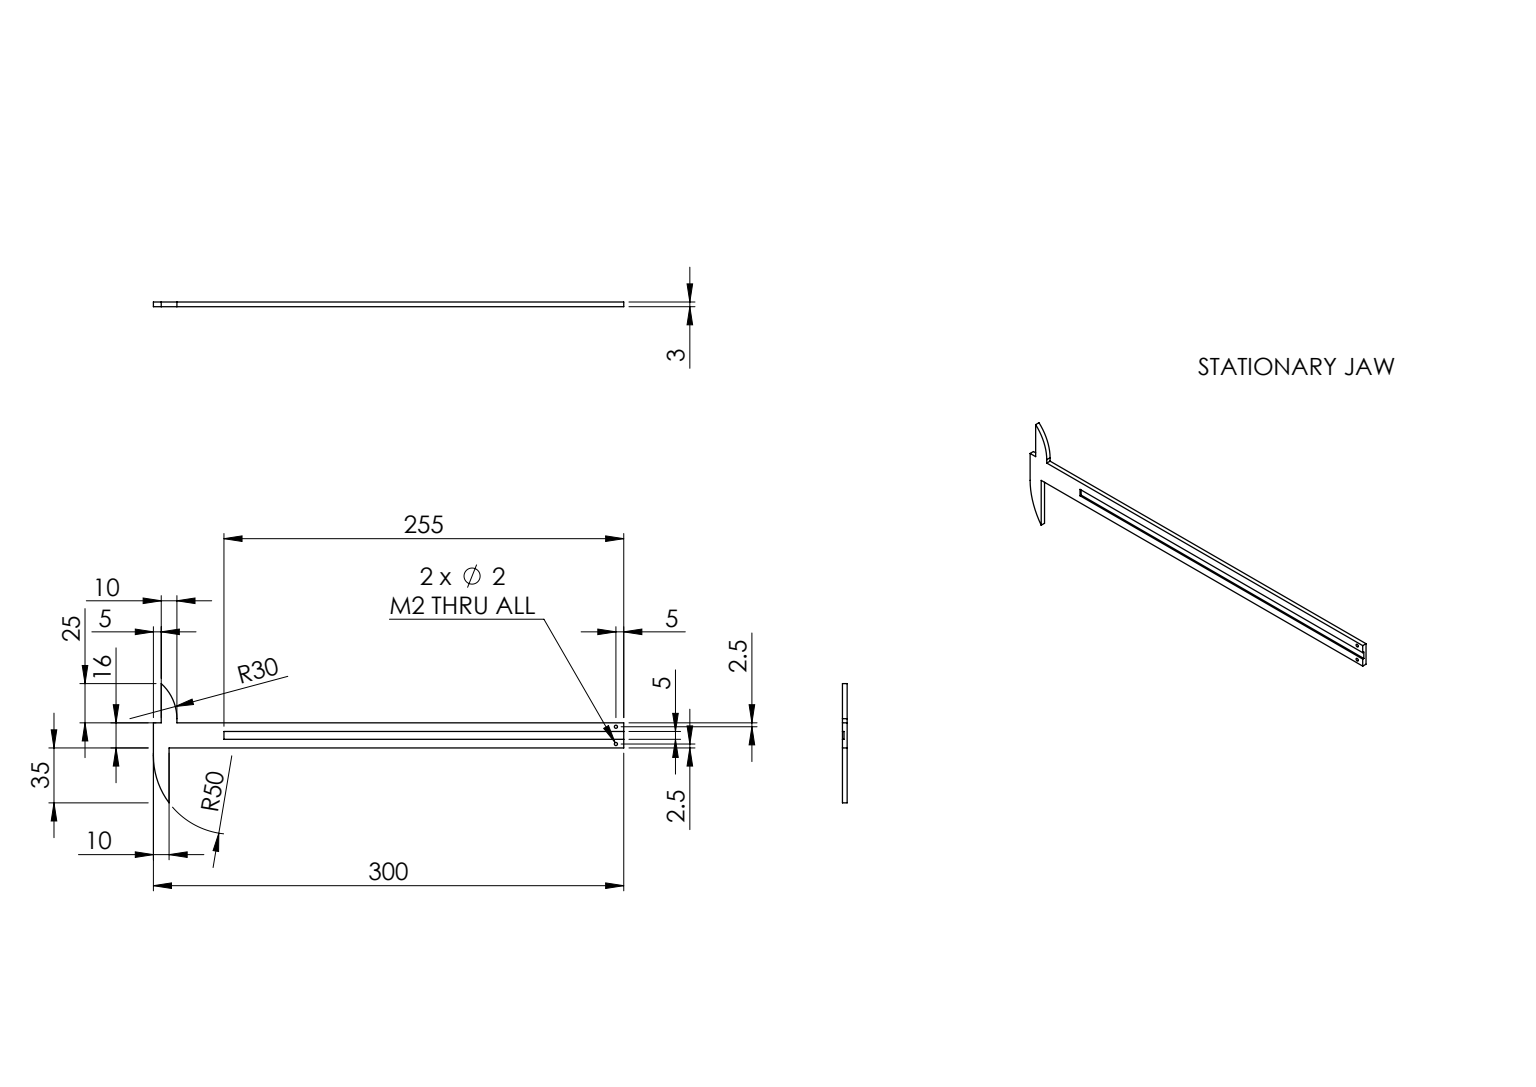
ISO-10303-21;
HEADER;
FILE_DESCRIPTION (('STEP AP214'),
    '1' );
FILE_NAME ('stationary jaw.step',
    '2026-10-27T04:40:18',
    ( '' ),
    ( '' ),
    'SwSTEP 2.0',
    'SolidWorks 2026',
    '' );
FILE_SCHEMA (( 'AUTOMOTIVE_DESIGN' ));
ENDSEC;

DATA;
#11=FACE_OUTER_BOUND ( 'NONE', #2535, .T. ) ;
#34=CARTESIAN_POINT ( 'NONE',  ( -149.9999999999999716, 8.000000000000000000, 0.000000000000000000 ) ) ;
#53=CARTESIAN_POINT ( 'NONE',  ( 144.0000000000000284, -5.500000000000000000, 3.000000000000000000 ) ) ;
#117=DIRECTION ( 'NONE',  ( 0.000000000000000000, 0.000000000000000000, 1.000000000000000000 ) ) ;
#146=EDGE_CURVE ( 'NONE', #6970, #9736, #4895, .T. ) ;
#150=VECTOR ( 'NONE', #8789, 1000.000000000000000 ) ;
#162=AXIS2_PLACEMENT_3D ( 'NONE', #9186, #3975, #9242 ) ;
#173=DIRECTION ( 'NONE',  ( -0.000000000000000000, -0.000000000000000000, 1.000000000000000000 ) ) ;
#192=VERTEX_POINT ( 'NONE', #7412 ) ;
#204=( NAMED_UNIT ( * ) PLANE_ANGLE_UNIT ( ) SI_UNIT ( $, .RADIAN. ) );
#247=ADVANCED_FACE ( 'NONE', ( #10016 ), #2398, .F. ) ;
#272=DIRECTION ( 'NONE',  ( 0.000000000000000000, 0.000000000000000000, -1.000000000000000000 ) ) ;
#276=DIRECTION ( 'NONE',  ( 1.000000000000000000, 0.000000000000000000, 0.000000000000000000 ) ) ;
#313=CARTESIAN_POINT ( 'NONE',  ( -105.0000000000000000, -2.500000000000000000, 4.000000000000000000 ) ) ;
#328=CIRCLE ( 'NONE', #5652, 1.000000000000000888 ) ;
#334=DIRECTION ( 'NONE',  ( 1.000000000000000000, 0.000000000000000000, 0.000000000000000000 ) ) ;
#362=EDGE_CURVE ( 'NONE', #4689, #5869, #2786, .T. ) ;
#386=VERTEX_POINT ( 'NONE', #1056 ) ;
#391=ORIENTED_EDGE ( 'NONE', *, *, #9319, .T. ) ;
#404=DIRECTION ( 'NONE',  ( 0.000000000000000000, 0.000000000000000000, 1.000000000000000000 ) ) ;
#406=DIRECTION ( 'NONE',  ( 1.734723475976807094E-15, -1.000000000000000000, 0.000000000000000000 ) ) ;
#407=UNCERTAINTY_MEASURE_WITH_UNIT (LENGTH_MEASURE( 1.000000000000000082E-05 ), #5246, 'distance_accuracy_value', 'NONE');
#409=EDGE_LOOP ( 'NONE', ( #9606, #6475, #9228, #1255, #10309, #5081, #6466, #4394, #2415, #6355, #391, #7202, #777, #5042 ) ) ;
#427=VERTEX_POINT ( 'NONE', #7181 ) ;
#477=CARTESIAN_POINT ( 'NONE',  ( 0.000000000000000000, -2.500000000000000000, 3.000000000000000000 ) ) ;
#478=ORIENTED_EDGE ( 'NONE', *, *, #3539, .T. ) ;
#503=ADVANCED_FACE ( 'NONE', ( #6406 ), #2069, .T. ) ;
#510=LINE ( 'NONE', #9841, #4674 ) ;
#547=AXIS2_PLACEMENT_3D ( 'NONE', #10152, #5041, #1715 ) ;
#567=CARTESIAN_POINT ( 'NONE',  ( -149.9999999999999716, 8.000000000000000000, 3.000000000000000000 ) ) ;
#573=DIRECTION ( 'NONE',  ( -0.000000000000000000, -0.000000000000000000, 1.000000000000000000 ) ) ;
#592=AXIS2_PLACEMENT_3D ( 'NONE', #10434, #7171, #272 ) ;
#599=AXIS2_PLACEMENT_3D ( 'NONE', #4517, #5230, #6973 ) ;
#604=CIRCLE ( 'NONE', #9648, 1.000000000000000888 ) ;
#667=LINE ( 'NONE', #7455, #4965 ) ;
#670=LINE ( 'NONE', #9229, #10699 ) ;
#678=AXIS2_PLACEMENT_3D ( 'NONE', #10292, #1697, #1916 ) ;
#680=DIRECTION ( 'NONE',  ( -0.000000000000000000, 1.000000000000000000, -0.000000000000000000 ) ) ;
#683=AXIS2_PLACEMENT_3D ( 'NONE', #6099, #5365, #6331 ) ;
#686=FACE_BOUND ( 'NONE', #7136, .T. ) ;
#687=CARTESIAN_POINT ( 'NONE',  ( 150.0000000000000284, -8.000000000000000000, 3.000000000000000000 ) ) ;
#725=DIRECTION ( 'NONE',  ( -1.734723475976807094E-15, 1.000000000000000000, 0.000000000000000000 ) ) ;
#727=DIRECTION ( 'NONE',  ( 1.110223024625156540E-15, 1.000000000000000000, 0.000000000000000000 ) ) ;
#730=CARTESIAN_POINT ( 'NONE',  ( -149.9999999999999716, -8.000000000000000000, 0.000000000000000000 ) ) ;
#731=CARTESIAN_POINT ( 'NONE',  ( -149.9999999999999716, 8.000000000000000000, 0.000000000000000000 ) ) ;
#738=EDGE_LOOP ( 'NONE', ( #3698, #10471 ) ) ;
#740=PLANE ( 'NONE',  #6798 ) ;
#762=DIRECTION ( 'NONE',  ( -1.734723475976807094E-15, 1.000000000000000000, 0.000000000000000000 ) ) ;
#767=VERTEX_POINT ( 'NONE', #4360 ) ;
#777=ORIENTED_EDGE ( 'NONE', *, *, #2224, .F. ) ;
#814=EDGE_LOOP ( 'NONE', ( #8407, #1313, #7773, #3216 ) ) ;
#844=VECTOR ( 'NONE', #7783, 1000.000000000000000 ) ;
#883=DIRECTION ( 'NONE',  ( -0.000000000000000000, -0.000000000000000000, 1.000000000000000000 ) ) ;
#891=ORIENTED_EDGE ( 'NONE', *, *, #2292, .T. ) ;
#922=( NAMED_UNIT ( * ) SI_UNIT ( $, .STERADIAN. ) SOLID_ANGLE_UNIT ( ) );
#943=EDGE_CURVE ( 'NONE', #5113, #386, #9778, .T. ) ;
#991=LINE ( 'NONE', #10159, #844 ) ;
#998=ORIENTED_EDGE ( 'NONE', *, *, #7274, .T. ) ;
#1006=ORIENTED_EDGE ( 'NONE', *, *, #5250, .T. ) ;
#1028=CARTESIAN_POINT ( 'NONE',  ( -134.9999999999999147, 8.000000000000000000, 0.000000000000000000 ) ) ;
#1033=ORIENTED_EDGE ( 'NONE', *, *, #9359, .T. ) ;
#1039=ORIENTED_EDGE ( 'NONE', *, *, #2073, .T. ) ;
#1041=COLOUR_RGB ( '',0.8941176470588234615, 0.8941176470588234615, 0.8941176470588234615 ) ;
#1056=CARTESIAN_POINT ( 'NONE',  ( -144.9999999999999432, 8.000000000000000000, 0.000000000000000000 ) ) ;
#1077=CARTESIAN_POINT ( 'NONE',  ( -134.9999999999999147, 10.63932022500203267, 3.000000000000000000 ) ) ;
#1084=ORIENTED_EDGE ( 'NONE', *, *, #7761, .F. ) ;
#1090=( NAMED_UNIT ( * ) PLANE_ANGLE_UNIT ( ) SI_UNIT ( $, .RADIAN. ) );
#1110=CARTESIAN_POINT ( 'NONE',  ( -139.9999999999999716, -43.00000000000000000, 3.000000000000000000 ) ) ;
#1153=ORIENTED_EDGE ( 'NONE', *, *, #10665, .F. ) ;
#1162=ORIENTED_EDGE ( 'NONE', *, *, #6843, .F. ) ;
#1170=UNCERTAINTY_MEASURE_WITH_UNIT (LENGTH_MEASURE( 1.000000000000000082E-05 ), #8148, 'distance_accuracy_value', 'NONE');
#1175=VERTEX_POINT ( 'NONE', #1533 ) ;
#1190=VERTEX_POINT ( 'NONE', #6192 ) ;
#1219=ADVANCED_FACE ( 'NONE', ( #8526 ), #8695, .F. ) ;
#1223=PLANE ( 'NONE',  #592 ) ;
#1227=CARTESIAN_POINT ( 'NONE',  ( -149.9999999999999716, -8.000000000000000000, 3.000000000000000000 ) ) ;
#1255=ORIENTED_EDGE ( 'NONE', *, *, #3655, .T. ) ;
#1280=EDGE_CURVE ( 'NONE', #10017, #2164, #4461, .T. ) ;
#1313=ORIENTED_EDGE ( 'NONE', *, *, #1429, .T. ) ;
#1317=EDGE_CURVE ( 'NONE', #4292, #7283, #10867, .T. ) ;
#1321=MANIFOLD_SOLID_BREP ( 'Cavity1', #4988 ) ;
#1322=ORIENTED_EDGE ( 'NONE', *, *, #943, .F. ) ;
#1334=FACE_OUTER_BOUND ( 'NONE', #6161, .T. ) ;
#1341=DIRECTION ( 'NONE',  ( -1.734723475976807094E-15, 1.000000000000000000, 0.000000000000000000 ) ) ;
#1369=( NAMED_UNIT ( * ) PLANE_ANGLE_UNIT ( ) SI_UNIT ( $, .RADIAN. ) );
#1420=LINE ( 'NONE', #7253, #4126 ) ;
#1429=EDGE_CURVE ( 'NONE', #7720, #9736, #1420, .T. ) ;
#1438=FACE_OUTER_BOUND ( 'NONE', #10048, .T. ) ;
#1482=AXIS2_PLACEMENT_3D ( 'NONE', #3684, #9465, #6135 ) ;
#1507=ADVANCED_FACE ( 'NONE', ( #8298 ), #740, .F. ) ;
#1533=CARTESIAN_POINT ( 'NONE',  ( 144.0000000000000284, -5.500000000000000000, 0.000000000000000000 ) ) ;
#1540=FACE_OUTER_BOUND ( 'NONE', #2254, .T. ) ;
#1568=VECTOR ( 'NONE', #334, 1000.000000000000000 ) ;
#1569=CARTESIAN_POINT ( 'NONE',  ( -149.9999999999999716, -8.000000000000000000, 3.000000000000000000 ) ) ;
#1570=ORIENTED_EDGE ( 'NONE', *, *, #9359, .F. ) ;
#1587=EDGE_CURVE ( 'NONE', #6091, #7156, #6797, .T. ) ;
#1596=ORIENTED_EDGE ( 'NONE', *, *, #943, .T. ) ;
#1627=CARTESIAN_POINT ( 'NONE',  ( -149.9999999999999716, 8.000000000000000000, 3.000000000000000000 ) ) ;
#1656=VECTOR ( 'NONE', #9806, 1000.000000000000000 ) ;
#1671=EDGE_CURVE ( 'NONE', #427, #10197, #5953, .T. ) ;
#1678=ADVANCED_FACE ( 'NONE', ( #1731 ), #3448, .F. ) ;
#1688=CARTESIAN_POINT ( 'NONE',  ( 146.0000000000000284, 5.500000000000000000, 0.000000000000000000 ) ) ;
#1697=DIRECTION ( 'NONE',  ( -0.000000000000000000, -0.000000000000000000, 1.000000000000000000 ) ) ;
#1703=LINE ( 'NONE', #34, #9038 ) ;
#1706=DIRECTION ( 'NONE',  ( 1.000000000000000000, 0.000000000000000000, 0.000000000000000000 ) ) ;
#1715=DIRECTION ( 'NONE',  ( -1.110223024625156343E-15, 1.000000000000000000, 0.000000000000000000 ) ) ;
#1717=LINE ( 'NONE', #6106, #5354 ) ;
#1731=FACE_OUTER_BOUND ( 'NONE', #7420, .T. ) ;
#1751=ORIENTED_EDGE ( 'NONE', *, *, #1280, .F. ) ;
#1760=DIRECTION ( 'NONE',  ( -0.000000000000000000, -0.000000000000000000, 1.000000000000000000 ) ) ;
#1774=EDGE_LOOP ( 'NONE', ( #7389, #6028, #6329, #3980 ) ) ;
#1779=EDGE_CURVE ( 'NONE', #5869, #2164, #8054, .T. ) ;
#1780=CARTESIAN_POINT ( 'NONE',  ( -105.0000000000000000, 2.500000000000000000, 4.000000000000000000 ) ) ;
#1833=AXIS2_PLACEMENT_3D ( 'NONE', #6481, #6309, #4794 ) ;
#1842=CARTESIAN_POINT ( 'NONE',  ( -105.0000000000000000, -2.500000000000000000, 2.000000000000000000 ) ) ;
#1858=CARTESIAN_POINT ( 'NONE',  ( 144.0000000000000284, 5.500000000000000000, 3.000000000000000000 ) ) ;
#1876=SURFACE_STYLE_USAGE ( .BOTH. , #10308 ) ;
#1889=CARTESIAN_POINT ( 'NONE',  ( -144.9999999999999716, 33.00000000000000000, 0.000000000000000000 ) ) ;
#1916=DIRECTION ( 'NONE',  ( 1.000000000000000000, 0.000000000000000000, 0.000000000000000000 ) ) ;
#1927=AXIS2_PLACEMENT_3D ( 'NONE', #10763, #3154, #2167 ) ;
#1936=AXIS2_PLACEMENT_3D ( 'NONE', #9363, #8538, #6708 ) ;
#1940=CARTESIAN_POINT ( 'NONE',  ( -149.9999999999999716, -12.99999999999998757, 0.000000000000000000 ) ) ;
#1942=ORIENTED_EDGE ( 'NONE', *, *, #10570, .F. ) ;
#1945=LINE ( 'NONE', #7670, #6987 ) ;
#1952=CARTESIAN_POINT ( 'NONE',  ( 145.0000000000000284, -5.500000000000000000, 0.000000000000000000 ) ) ;
#1998=CARTESIAN_POINT ( 'NONE',  ( -105.0000000000000000, 2.500000000000000000, 2.000000000000000000 ) ) ;
#2005=CARTESIAN_POINT ( 'NONE',  ( 145.0000000000000284, -5.500000000000000000, 3.000000000000000000 ) ) ;
#2006=VECTOR ( 'NONE', #117, 1000.000000000000000 ) ;
#2062=CARTESIAN_POINT ( 'NONE',  ( -139.9999999999999716, -43.00000000000000000, 3.000000000000000000 ) ) ;
#2069=CYLINDRICAL_SURFACE ( 'NONE', #8218, 30.00000000000000000 ) ;
#2073=EDGE_CURVE ( 'NONE', #427, #7723, #5227, .T. ) ;
#2103=EDGE_CURVE ( 'NONE', #9392, #1175, #604, .T. ) ;
#2114=ORIENTED_EDGE ( 'NONE', *, *, #2619, .T. ) ;
#2115=DIRECTION ( 'NONE',  ( 0.000000000000000000, -1.000000000000000000, 0.000000000000000000 ) ) ;
#2127=EDGE_LOOP ( 'NONE', ( #10724, #4904, #5313, #1006 ) ) ;
#2157=CARTESIAN_POINT ( 'NONE',  ( -134.9999999999999147, 8.000000000000000000, 3.000000000000000000 ) ) ;
#2164=VERTEX_POINT ( 'NONE', #1858 ) ;
#2167=DIRECTION ( 'NONE',  ( 0.000000000000000000, -0.000000000000000000, -1.000000000000000000 ) ) ;
#2176=LINE ( 'NONE', #567, #4928 ) ;
#2182=VECTOR ( 'NONE', #727, 1000.000000000000000 ) ;
#2189=AXIS2_PLACEMENT_3D ( 'NONE', #6956, #9339, #10337 ) ;
#2224=EDGE_CURVE ( 'NONE', #192, #2429, #7198, .T. ) ;
#2225=ORIENTED_EDGE ( 'NONE', *, *, #10290, .T. ) ;
#2231=CARTESIAN_POINT ( 'NONE',  ( 150.0000000000000000, 8.000000000000000000, 3.000000000000000000 ) ) ;
#2234=VERTEX_POINT ( 'NONE', #4687 ) ;
#2252=CARTESIAN_POINT ( 'NONE',  ( 146.0000000000000284, -5.500000000000000000, 3.000000000000000000 ) ) ;
#2254=EDGE_LOOP ( 'NONE', ( #1322, #9808, #4811, #8979, #8645, #4632, #1942, #4154, #7191, #4501 ) ) ;
#2266=EDGE_CURVE ( 'NONE', #5113, #7871, #5189, .T. ) ;
#2292=EDGE_CURVE ( 'NONE', #9531, #2234, #5579, .T. ) ;
#2307=AXIS2_PLACEMENT_3D ( 'NONE', #5193, #3646, #1706 ) ;
#2321=CARTESIAN_POINT ( 'NONE',  ( 144.0000000000000284, 5.500000000000000000, 0.000000000000000000 ) ) ;
#2398=PLANE ( 'NONE',  #5534 ) ;
#2415=ORIENTED_EDGE ( 'NONE', *, *, #7985, .T. ) ;
#2422=CARTESIAN_POINT ( 'NONE',  ( -99.99999999999995737, -12.99999999999998757, 3.000000000000000000 ) ) ;
#2429=VERTEX_POINT ( 'NONE', #6630 ) ;
#2437=AXIS2_PLACEMENT_3D ( 'NONE', #7643, #10183, #3463 ) ;
#2447=CARTESIAN_POINT ( 'NONE',  ( -139.9999999999999716, -8.000000000000000000, 0.000000000000000000 ) ) ;
#2482=AXIS2_PLACEMENT_3D ( 'NONE', #2422, #2591, #5928 ) ;
#2492=DIRECTION ( 'NONE',  ( 0.000000000000000000, 0.000000000000000000, -1.000000000000000000 ) ) ;
#2502=DIRECTION ( 'NONE',  ( 0.000000000000000000, -0.000000000000000000, -1.000000000000000000 ) ) ;
#2535=EDGE_LOOP ( 'NONE', ( #10120, #10464, #891, #8479 ) ) ;
#2544=LINE ( 'NONE', #5933, #5989 ) ;
#2563=DIRECTION ( 'NONE',  ( -0.000000000000000000, -0.000000000000000000, 1.000000000000000000 ) ) ;
#2591=DIRECTION ( 'NONE',  ( -0.000000000000000000, -0.000000000000000000, 1.000000000000000000 ) ) ;
#2598=SHAPE_DEFINITION_REPRESENTATION ( #4206, #5016 ) ;
#2612=CARTESIAN_POINT ( 'NONE',  ( -144.9999999999999716, 33.00000000000000000, 3.000000000000000000 ) ) ;
#2619=EDGE_CURVE ( 'NONE', #10003, #386, #1945, .T. ) ;
#2651=DIRECTION ( 'NONE',  ( 0.000000000000000000, 1.000000000000000000, 0.000000000000000000 ) ) ;
#2663=DIRECTION ( 'NONE',  ( 0.000000000000000000, -1.000000000000000000, 0.000000000000000000 ) ) ;
#2667=EDGE_CURVE ( 'NONE', #1175, #3747, #9383, .T. ) ;
#2714=PLANE ( 'NONE',  #683 ) ;
#2748=EDGE_LOOP ( 'NONE', ( #7649, #3570, #5654, #3760 ) ) ;
#2749=CARTESIAN_POINT ( 'NONE',  ( 144.0000000000000284, 5.500000000000000000, 3.000000000000000000 ) ) ;
#2786=LINE ( 'NONE', #5104, #9426 ) ;
#2825=AXIS2_PLACEMENT_3D ( 'NONE', #4035, #6451, #6557 ) ;
#2830=EDGE_CURVE ( 'NONE', #9377, #9531, #510, .T. ) ;
#2831=VECTOR ( 'NONE', #9134, 1000.000000000000000 ) ;
#2833=DIRECTION ( 'NONE',  ( 1.110223024625156540E-15, -1.000000000000000000, -0.000000000000000000 ) ) ;
#2879=FACE_OUTER_BOUND ( 'NONE', #10873, .T. ) ;
#2893=CIRCLE ( 'NONE', #3776, 1.000000000000000888 ) ;
#2918=EDGE_CURVE ( 'NONE', #6183, #2234, #6759, .T. ) ;
#2921=VECTOR ( 'NONE', #8474, 1000.000000000000000 ) ;
#2955=CARTESIAN_POINT ( 'NONE',  ( -139.9999999999999716, -8.000000000000000000, 3.000000000000000000 ) ) ;
#2975=CARTESIAN_POINT ( 'NONE',  ( -149.9999999999999716, -8.000000000000000000, 0.000000000000000000 ) ) ;
#2978=( NAMED_UNIT ( * ) SI_UNIT ( $, .STERADIAN. ) SOLID_ANGLE_UNIT ( ) );
#2992=DIRECTION ( 'NONE',  ( 0.000000000000000000, 0.000000000000000000, 1.000000000000000000 ) ) ;
#2994=VERTEX_POINT ( 'NONE', #9356 ) ;
#3005=VECTOR ( 'NONE', #680, 1000.000000000000000 ) ;
#3018=AXIS2_PLACEMENT_3D ( 'NONE', #10948, #173, #10335 ) ;
#3047=FACE_OUTER_BOUND ( 'NONE', #2127, .T. ) ;
#3071=CARTESIAN_POINT ( 'NONE',  ( 145.0000000000000284, 5.500000000000000000, 3.000000000000000000 ) ) ;
#3087=EDGE_CURVE ( 'NONE', #7723, #1190, #3467, .T. ) ;
#3114=CARTESIAN_POINT ( 'NONE',  ( -139.9999999999999716, -8.000000000000000000, 0.000000000000000000 ) ) ;
#3126=CARTESIAN_POINT ( 'NONE',  ( 150.0000000000000284, -2.500000000000000000, 2.000000000000000000 ) ) ;
#3138=DIRECTION ( 'NONE',  ( 0.000000000000000000, -0.000000000000000000, 1.000000000000000000 ) ) ;
#3154=DIRECTION ( 'NONE',  ( 0.000000000000000000, -1.000000000000000000, 0.000000000000000000 ) ) ;
#3216=ORIENTED_EDGE ( 'NONE', *, *, #6767, .T. ) ;
#3233=PLANE ( 'NONE',  #162 ) ;
#3261=FACE_BOUND ( 'NONE', #3740, .T. ) ;
#3266=EDGE_LOOP ( 'NONE', ( #5242, #10695, #6445, #4094 ) ) ;
#3298=ORIENTED_EDGE ( 'NONE', *, *, #6350, .F. ) ;
#3309=CARTESIAN_POINT ( 'NONE',  ( 150.0000000000000000, 8.000000000000000000, 3.000000000000000000 ) ) ;
#3328=DIRECTION ( 'NONE',  ( 0.000000000000000000, -1.000000000000000000, 0.000000000000000000 ) ) ;
#3344=VECTOR ( 'NONE', #5947, 1000.000000000000000 ) ;
#3353=CIRCLE ( 'NONE', #10258, 1.000000000000000888 ) ;
#3358=ADVANCED_FACE ( 'NONE', ( #9036 ), #9143, .T. ) ;
#3385=LINE ( 'NONE', #9388, #8161 ) ;
#3418=DIRECTION ( 'NONE',  ( -1.000000000000000000, -0.000000000000000000, -0.000000000000000000 ) ) ;
#3448=CYLINDRICAL_SURFACE ( 'NONE', #2189, 1.000000000000000888 ) ;
#3463=DIRECTION ( 'NONE',  ( 1.000000000000000000, 0.000000000000000000, 0.000000000000000000 ) ) ;
#3467=LINE ( 'NONE', #5712, #9830 ) ;
#3529=ORIENTED_EDGE ( 'NONE', *, *, #2224, .T. ) ;
#3539=EDGE_CURVE ( 'NONE', #1175, #9392, #3353, .T. ) ;
#3541=ORIENTED_EDGE ( 'NONE', *, *, #10290, .F. ) ;
#3570=ORIENTED_EDGE ( 'NONE', *, *, #4304, .T. ) ;
#3643=PLANE ( 'NONE',  #8876 ) ;
#3646=DIRECTION ( 'NONE',  ( 0.000000000000000000, 0.000000000000000000, 1.000000000000000000 ) ) ;
#3655=EDGE_CURVE ( 'NONE', #7156, #4292, #5777, .T. ) ;
#3661=LINE ( 'NONE', #1227, #1568 ) ;
#3684=CARTESIAN_POINT ( 'NONE',  ( -164.9999999999999147, 10.63932022500206642, 3.000000000000000000 ) ) ;
#3698=ORIENTED_EDGE ( 'NONE', *, *, #6843, .T. ) ;
#3714=( GEOMETRIC_REPRESENTATION_CONTEXT ( 3 ) GLOBAL_UNCERTAINTY_ASSIGNED_CONTEXT ( ( #407 ) ) GLOBAL_UNIT_ASSIGNED_CONTEXT ( ( #5246, #1090, #922 ) ) REPRESENTATION_CONTEXT ( 'NONE', 'WORKASPACE' ) );
#3727=DIRECTION ( 'NONE',  ( 1.000000000000000000, 0.000000000000000000, 0.000000000000000000 ) ) ;
#3735=EDGE_LOOP ( 'NONE', ( #10063, #3849, #10923, #8656 ) ) ;
#3740=EDGE_LOOP ( 'NONE', ( #4279, #478 ) ) ;
#3747=VERTEX_POINT ( 'NONE', #10007 ) ;
#3757=EDGE_CURVE ( 'NONE', #6540, #7871, #670, .T. ) ;
#3760=ORIENTED_EDGE ( 'NONE', *, *, #10548, .T. ) ;
#3762=CARTESIAN_POINT ( 'NONE',  ( -105.0000000000000000, 2.500000000000000000, 3.000000000000000000 ) ) ;
#3767=ORIENTED_EDGE ( 'NONE', *, *, #2619, .F. ) ;
#3776=AXIS2_PLACEMENT_3D ( 'NONE', #5552, #6665, #9945 ) ;
#3824=EDGE_CURVE ( 'NONE', #6498, #192, #1717, .T. ) ;
#3849=ORIENTED_EDGE ( 'NONE', *, *, #9213, .T. ) ;
#3908=CARTESIAN_POINT ( 'NONE',  ( -134.9999999999999147, 8.000000000000000000, 3.000000000000000000 ) ) ;
#3930=DIRECTION ( 'NONE',  ( -1.000000000000000000, 0.000000000000000000, 0.000000000000000000 ) ) ;
#3932=ADVANCED_FACE ( 'NONE', ( #10495 ), #8007, .F. ) ;
#3940=ADVANCED_FACE ( 'NONE', ( #7116 ), #1223, .F. ) ;
#3946=DIRECTION ( 'NONE',  ( -1.000000000000000000, -0.000000000000000000, -0.000000000000000000 ) ) ;
#3975=DIRECTION ( 'NONE',  ( 0.000000000000000000, 0.000000000000000000, -1.000000000000000000 ) ) ;
#3980=ORIENTED_EDGE ( 'NONE', *, *, #10692, .F. ) ;
#3983=DIRECTION ( 'NONE',  ( 1.000000000000000000, 0.000000000000000000, 0.000000000000000000 ) ) ;
#4035=CARTESIAN_POINT ( 'NONE',  ( 145.0000000000000284, 5.500000000000000000, 3.000000000000000000 ) ) ;
#4038=EDGE_CURVE ( 'NONE', #10017, #4689, #2893, .T. ) ;
#4094=ORIENTED_EDGE ( 'NONE', *, *, #362, .F. ) ;
#4126=VECTOR ( 'NONE', #3138, 1000.000000000000000 ) ;
#4154=ORIENTED_EDGE ( 'NONE', *, *, #9639, .T. ) ;
#4188=CARTESIAN_POINT ( 'NONE',  ( 150.0000000000000284, 2.500000000000000000, 3.000000000000000000 ) ) ;
#4205=AXIS2_PLACEMENT_3D ( 'NONE', #1780, #3328, #2502 ) ;
#4206=PRODUCT_DEFINITION_SHAPE ( 'NONE', 'NONE',  #10302 ) ;
#4215=CARTESIAN_POINT ( 'NONE',  ( -105.0000000000000000, 2.500000000000000000, 4.000000000000000000 ) ) ;
#4249=FILL_AREA_STYLE_COLOUR ( '', #1041 ) ;
#4267=LINE ( 'NONE', #4215, #3344 ) ;
#4268=LINE ( 'NONE', #2612, #7441 ) ;
#4279=ORIENTED_EDGE ( 'NONE', *, *, #2103, .T. ) ;
#4292=VERTEX_POINT ( 'NONE', #1077 ) ;
#4299=FACE_BOUND ( 'NONE', #738, .T. ) ;
#4301=AXIS2_PLACEMENT_3D ( 'NONE', #3071, #573, #7129 ) ;
#4304=EDGE_CURVE ( 'NONE', #7871, #4292, #10235, .T. ) ;
#4323=LINE ( 'NONE', #1842, #7979 ) ;
#4350=DIRECTION ( 'NONE',  ( 0.000000000000000000, -0.000000000000000000, 1.000000000000000000 ) ) ;
#4357=DIRECTION ( 'NONE',  ( -0.000000000000000000, -0.000000000000000000, -1.000000000000000000 ) ) ;
#4360=CARTESIAN_POINT ( 'NONE',  ( 150.0000000000000000, 8.000000000000000000, 0.000000000000000000 ) ) ;
#4394=ORIENTED_EDGE ( 'NONE', *, *, #146, .T. ) ;
#4403=ORIENTED_EDGE ( 'NONE', *, *, #10665, .T. ) ;
#4419=FILL_AREA_STYLE ('',( #4249 ) ) ;
#4461=LINE ( 'NONE', #2749, #10525 ) ;
#4465=DIRECTION ( 'NONE',  ( 0.000000000000000000, 0.000000000000000000, 1.000000000000000000 ) ) ;
#4500=DIRECTION ( 'NONE',  ( 1.000000000000000000, 0.000000000000000000, 0.000000000000000000 ) ) ;
#4501=ORIENTED_EDGE ( 'NONE', *, *, #6269, .F. ) ;
#4517=CARTESIAN_POINT ( 'NONE',  ( 145.0000000000000284, -5.500000000000000000, 3.000000000000000000 ) ) ;
#4536=CARTESIAN_POINT ( 'NONE',  ( -149.9999999999999716, -12.99999999999998757, 3.000000000000000000 ) ) ;
#4549=DIRECTION ( 'NONE',  ( -0.000000000000000000, -0.000000000000000000, 1.000000000000000000 ) ) ;
#4587=VECTOR ( 'NONE', #7705, 1000.000000000000000 ) ;
#4600=ORIENTED_EDGE ( 'NONE', *, *, #5877, .T. ) ;
#4632=ORIENTED_EDGE ( 'NONE', *, *, #2292, .F. ) ;
#4663=DIRECTION ( 'NONE',  ( -0.000000000000000000, -0.000000000000000000, -1.000000000000000000 ) ) ;
#4672=DIRECTION ( 'NONE',  ( 0.000000000000000000, 1.000000000000000000, 0.000000000000000000 ) ) ;
#4674=VECTOR ( 'NONE', #10556, 1000.000000000000000 ) ;
#4687=CARTESIAN_POINT ( 'NONE',  ( 150.0000000000000284, -8.000000000000000000, 0.000000000000000000 ) ) ;
#4689=VERTEX_POINT ( 'NONE', #1688 ) ;
#4694=ORIENTED_EDGE ( 'NONE', *, *, #7985, .F. ) ;
#4698=LINE ( 'NONE', #2447, #3005 ) ;
#4704=ORIENTED_EDGE ( 'NONE', *, *, #9696, .F. ) ;
#4712=ORIENTED_EDGE ( 'NONE', *, *, #2266, .F. ) ;
#4723=ORIENTED_EDGE ( 'NONE', *, *, #3087, .T. ) ;
#4794=DIRECTION ( 'NONE',  ( -1.000000000000000000, 0.000000000000000000, 0.000000000000000000 ) ) ;
#4806=CARTESIAN_POINT ( 'NONE',  ( -105.0000000000000000, -2.500000000000000000, 4.000000000000000000 ) ) ;
#4811=ORIENTED_EDGE ( 'NONE', *, *, #3757, .F. ) ;
#4814=PLANE ( 'NONE',  #1927 ) ;
#4822=DIRECTION ( 'NONE',  ( -0.000000000000000000, -1.000000000000000000, -0.000000000000000000 ) ) ;
#4826=VECTOR ( 'NONE', #2833, 1000.000000000000000 ) ;
#4853=APPLICATION_CONTEXT ( 'automotive_design' ) ;
#4895=LINE ( 'NONE', #1569, #7147 ) ;
#4896=EDGE_LOOP ( 'NONE', ( #8275, #9624, #4712, #4971 ) ) ;
#4897=DIRECTION ( 'NONE',  ( -0.000000000000000000, -0.000000000000000000, 1.000000000000000000 ) ) ;
#4904=ORIENTED_EDGE ( 'NONE', *, *, #2830, .F. ) ;
#4928=VECTOR ( 'NONE', #3946, 1000.000000000000000 ) ;
#4965=VECTOR ( 'NONE', #725, 1000.000000000000000 ) ;
#4971=ORIENTED_EDGE ( 'NONE', *, *, #5725, .F. ) ;
#4976=VERTEX_POINT ( 'NONE', #3126 ) ;
#4979=CARTESIAN_POINT ( 'NONE',  ( -134.9999999999999147, 10.63932022500203267, 3.000000000000000000 ) ) ;
#4985=EDGE_CURVE ( 'NONE', #9045, #7720, #6582, .T. ) ;
#4988=CLOSED_SHELL ( 'NONE', ( #6211, #1678, #1507, #6707, #9980, #3932, #3940, #7044, #6382, #8331, #7429, #9732, #8443, #503, #1219, #8713, #247, #9188, #3358, #6497 ) ) ;
#5016=SHAPE_REPRESENTATION ( 'stationary jaw', ( #2307 ), #3714 ) ;
#5036=CARTESIAN_POINT ( 'NONE',  ( -99.99999999999995737, -12.99999999999998757, 0.000000000000000000 ) ) ;
#5041=DIRECTION ( 'NONE',  ( 1.000000000000000000, 1.110223024625156343E-15, -0.000000000000000000 ) ) ;
#5042=ORIENTED_EDGE ( 'NONE', *, *, #3824, .F. ) ;
#5081=ORIENTED_EDGE ( 'NONE', *, *, #10917, .T. ) ;
#5104=CARTESIAN_POINT ( 'NONE',  ( 146.0000000000000284, 5.500000000000000000, 3.000000000000000000 ) ) ;
#5113=VERTEX_POINT ( 'NONE', #1889 ) ;
#5142=DIRECTION ( 'NONE',  ( -1.000000000000000000, 0.000000000000000000, 0.000000000000000000 ) ) ;
#5143=PRODUCT_CONTEXT ( 'NONE', #10872, 'mechanical' ) ;
#5189=CIRCLE ( 'NONE', #1833, 30.00000000000000000 ) ;
#5193=CARTESIAN_POINT ( 'NONE',  ( 0.000000000000000000, 0.000000000000000000, 0.000000000000000000 ) ) ;
#5194=ORIENTED_EDGE ( 'NONE', *, *, #2918, .T. ) ;
#5227=LINE ( 'NONE', #7748, #8762 ) ;
#5230=DIRECTION ( 'NONE',  ( -0.000000000000000000, -0.000000000000000000, 1.000000000000000000 ) ) ;
#5233=CYLINDRICAL_SURFACE ( 'NONE', #2437, 1.000000000000000888 ) ;
#5242=ORIENTED_EDGE ( 'NONE', *, *, #4038, .F. ) ;
#5246=( LENGTH_UNIT ( ) NAMED_UNIT ( * ) SI_UNIT ( .MILLI., .METRE. ) );
#5249=LINE ( 'NONE', #7163, #5820 ) ;
#5250=EDGE_CURVE ( 'NONE', #9380, #5859, #7174, .T. ) ;
#5313=ORIENTED_EDGE ( 'NONE', *, *, #9837, .F. ) ;
#5354=VECTOR ( 'NONE', #2663, 1000.000000000000000 ) ;
#5365=DIRECTION ( 'NONE',  ( -1.000000000000000000, 1.110223024625156343E-15, 0.000000000000000000 ) ) ;
#5479=EDGE_LOOP ( 'NONE', ( #1596, #3767, #9870, #9991 ) ) ;
#5482=DIRECTION ( 'NONE',  ( -0.000000000000000000, 1.000000000000000000, -0.000000000000000000 ) ) ;
#5487=LINE ( 'NONE', #7050, #7287 ) ;
#5499=PRODUCT_DEFINITION_FORMATION_WITH_SPECIFIED_SOURCE ( 'ANY', '', #7328, .NOT_KNOWN. ) ;
#5519=DIRECTION ( 'NONE',  ( 1.000000000000000000, 0.000000000000000000, 0.000000000000000000 ) ) ;
#5531=DIRECTION ( 'NONE',  ( -0.000000000000000000, -0.000000000000000000, -1.000000000000000000 ) ) ;
#5534=AXIS2_PLACEMENT_3D ( 'NONE', #5789, #5950, #8675 ) ;
#5552=CARTESIAN_POINT ( 'NONE',  ( 145.0000000000000284, 5.500000000000000000, 0.000000000000000000 ) ) ;
#5565=LINE ( 'NONE', #8963, #9769 ) ;
#5579=LINE ( 'NONE', #2975, #10339 ) ;
#5604=PRODUCT_DEFINITION_CONTEXT ( 'detailed design', #4853, 'design' ) ;
#5652=AXIS2_PLACEMENT_3D ( 'NONE', #2005, #7898, #276 ) ;
#5654=ORIENTED_EDGE ( 'NONE', *, *, #3655, .F. ) ;
#5668=MECHANICAL_DESIGN_GEOMETRIC_PRESENTATION_REPRESENTATION('',(#9935),#5839);
#5712=CARTESIAN_POINT ( 'NONE',  ( -105.0000000000000000, -2.500000000000000000, 2.000000000000000000 ) ) ;
#5725=EDGE_CURVE ( 'NONE', #7283, #5113, #4268, .T. ) ;
#5727=MECHANICAL_DESIGN_GEOMETRIC_PRESENTATION_REPRESENTATION('',(#7331),#8386);
#5777=LINE ( 'NONE', #3908, #2182 ) ;
#5789=CARTESIAN_POINT ( 'NONE',  ( 0.000000000000000000, 0.000000000000000000, 2.000000000000000000 ) ) ;
#5812=CARTESIAN_POINT ( 'NONE',  ( 150.0000000000000284, -8.000000000000000000, 3.000000000000000000 ) ) ;
#5820=VECTOR ( 'NONE', #5482, 1000.000000000000000 ) ;
#5833=CIRCLE ( 'NONE', #6729, 1.000000000000000888 ) ;
#5839=( GEOMETRIC_REPRESENTATION_CONTEXT ( 3 ) GLOBAL_UNCERTAINTY_ASSIGNED_CONTEXT ( ( #9733 ) ) GLOBAL_UNIT_ASSIGNED_CONTEXT ( ( #5978, #204, #9536 ) ) REPRESENTATION_CONTEXT ( 'NONE', 'WORKASPACE' ) );
#5845=LINE ( 'NONE', #1627, #2831 ) ;
#5859=VERTEX_POINT ( 'NONE', #9445 ) ;
#5869=VERTEX_POINT ( 'NONE', #9238 ) ;
#5877=EDGE_CURVE ( 'NONE', #1190, #4976, #4323, .T. ) ;
#5928=DIRECTION ( 'NONE',  ( -1.000000000000000000, 0.000000000000000000, 0.000000000000000000 ) ) ;
#5933=CARTESIAN_POINT ( 'NONE',  ( -105.0000000000000000, -2.500000000000000000, 4.000000000000000000 ) ) ;
#5947=DIRECTION ( 'NONE',  ( -0.000000000000000000, -0.000000000000000000, -1.000000000000000000 ) ) ;
#5948=DIRECTION ( 'NONE',  ( 1.000000000000000000, 0.000000000000000000, 0.000000000000000000 ) ) ;
#5950=DIRECTION ( 'NONE',  ( 0.000000000000000000, 0.000000000000000000, -1.000000000000000000 ) ) ;
#5952=PLANE ( 'NONE',  #6742 ) ;
#5953=LINE ( 'NONE', #9505, #2006 ) ;
#5967=EDGE_LOOP ( 'NONE', ( #8547, #7012, #1153, #1084, #5194, #998, #3541, #8117 ) ) ;
#5974=LINE ( 'NONE', #5812, #10451 ) ;
#5978=( LENGTH_UNIT ( ) NAMED_UNIT ( * ) SI_UNIT ( .MILLI., .METRE. ) );
#5989=VECTOR ( 'NONE', #4357, 1000.000000000000000 ) ;
#6000=DIRECTION ( 'NONE',  ( -0.000000000000000000, -0.000000000000000000, -1.000000000000000000 ) ) ;
#6028=ORIENTED_EDGE ( 'NONE', *, *, #9696, .T. ) ;
#6091=VERTEX_POINT ( 'NONE', #2231 ) ;
#6099=CARTESIAN_POINT ( 'NONE',  ( -134.9999999999999147, 8.000000000000000000, 3.000000000000000000 ) ) ;
#6106=CARTESIAN_POINT ( 'NONE',  ( -105.0000000000000000, 0.000000000000000000, 3.000000000000000000 ) ) ;
#6135=DIRECTION ( 'NONE',  ( -1.000000000000000000, 1.792547591842700533E-15, 0.000000000000000000 ) ) ;
#6161=EDGE_LOOP ( 'NONE', ( #4694, #8313, #9571, #6764 ) ) ;
#6164=DIRECTION ( 'NONE',  ( -0.000000000000000000, -0.000000000000000000, -1.000000000000000000 ) ) ;
#6183=VERTEX_POINT ( 'NONE', #8280 ) ;
#6192=CARTESIAN_POINT ( 'NONE',  ( -105.0000000000000000, -2.500000000000000000, 2.000000000000000000 ) ) ;
#6211=ADVANCED_FACE ( 'NONE', ( #7279 ), #10662, .F. ) ;
#6269=EDGE_CURVE ( 'NONE', #386, #9045, #1703, .T. ) ;
#6271=EDGE_LOOP ( 'NONE', ( #1039, #4723, #4600, #8149 ) ) ;
#6309=DIRECTION ( 'NONE',  ( 0.000000000000000000, 0.000000000000000000, -1.000000000000000000 ) ) ;
#6324=ORIENTED_EDGE ( 'NONE', *, *, #2667, .T. ) ;
#6329=ORIENTED_EDGE ( 'NONE', *, *, #3087, .F. ) ;
#6331=DIRECTION ( 'NONE',  ( -1.110223024625156343E-15, -1.000000000000000000, 0.000000000000000000 ) ) ;
#6347=CARTESIAN_POINT ( 'NONE',  ( -134.9999999999999147, 8.000000000000000000, 3.000000000000000000 ) ) ;
#6349=AXIS2_PLACEMENT_3D ( 'NONE', #9826, #10485, #10594 ) ;
#6350=EDGE_CURVE ( 'NONE', #3747, #2994, #5833, .T. ) ;
#6355=ORIENTED_EDGE ( 'NONE', *, *, #9837, .T. ) ;
#6382=ADVANCED_FACE ( 'NONE', ( #4299, #3261, #1540 ), #9155, .T. ) ;
#6389=CIRCLE ( 'NONE', #3018, 1.000000000000000888 ) ;
#6406=FACE_OUTER_BOUND ( 'NONE', #4896, .T. ) ;
#6408=EDGE_CURVE ( 'NONE', #10197, #6091, #5974, .T. ) ;
#6428=ORIENTED_EDGE ( 'NONE', *, *, #2103, .F. ) ;
#6445=ORIENTED_EDGE ( 'NONE', *, *, #8679, .T. ) ;
#6451=DIRECTION ( 'NONE',  ( -0.000000000000000000, -0.000000000000000000, 1.000000000000000000 ) ) ;
#6454=CARTESIAN_POINT ( 'NONE',  ( -134.9999999999999147, 10.63932022500203267, 0.000000000000000000 ) ) ;
#6465=CARTESIAN_POINT ( 'NONE',  ( -164.9999999999999147, 10.63932022500206642, 3.000000000000000000 ) ) ;
#6466=ORIENTED_EDGE ( 'NONE', *, *, #9482, .T. ) ;
#6475=ORIENTED_EDGE ( 'NONE', *, *, #6408, .T. ) ;
#6481=CARTESIAN_POINT ( 'NONE',  ( -164.9999999999999147, 10.63932022500206642, 0.000000000000000000 ) ) ;
#6494=PLANE ( 'NONE',  #9352 ) ;
#6497=ADVANCED_FACE ( 'NONE', ( #2879 ), #3643, .T. ) ;
#6498=VERTEX_POINT ( 'NONE', #3762 ) ;
#6524=ORIENTED_EDGE ( 'NONE', *, *, #10548, .F. ) ;
#6533=ORIENTED_EDGE ( 'NONE', *, *, #2667, .F. ) ;
#6540=VERTEX_POINT ( 'NONE', #1028 ) ;
#6551=ADVANCED_BREP_SHAPE_REPRESENTATION ( '', ( #1321, #2307 ), #3714 ) ;
#6557=DIRECTION ( 'NONE',  ( 1.000000000000000000, 0.000000000000000000, 0.000000000000000000 ) ) ;
#6559=LINE ( 'NONE', #9105, #7278 ) ;
#6582=LINE ( 'NONE', #730, #10075 ) ;
#6630=CARTESIAN_POINT ( 'NONE',  ( 150.0000000000000284, -2.500000000000000000, 3.000000000000000000 ) ) ;
#6643=CARTESIAN_POINT ( 'NONE',  ( -149.9999999999999716, 8.000000000000000000, 3.000000000000000000 ) ) ;
#6665=DIRECTION ( 'NONE',  ( -0.000000000000000000, -0.000000000000000000, 1.000000000000000000 ) ) ;
#6675=DIRECTION ( 'NONE',  ( 1.110223024625156540E-15, 1.000000000000000000, 0.000000000000000000 ) ) ;
#6707=ADVANCED_FACE ( 'NONE', ( #686, #10748, #7471 ), #3233, .F. ) ;
#6708=DIRECTION ( 'NONE',  ( -1.000000000000000000, 0.000000000000000000, -0.000000000000000000 ) ) ;
#6711=EDGE_CURVE ( 'NONE', #9392, #2994, #9969, .T. ) ;
#6722=ORIENTED_EDGE ( 'NONE', *, *, #362, .T. ) ;
#6729=AXIS2_PLACEMENT_3D ( 'NONE', #6763, #1760, #7488 ) ;
#6742=AXIS2_PLACEMENT_3D ( 'NONE', #9393, #4672, #8081 ) ;
#6759=LINE ( 'NONE', #10237, #2921 ) ;
#6763=CARTESIAN_POINT ( 'NONE',  ( 145.0000000000000284, -5.500000000000000000, 3.000000000000000000 ) ) ;
#6764=ORIENTED_EDGE ( 'NONE', *, *, #5250, .F. ) ;
#6767=EDGE_CURVE ( 'NONE', #6970, #9045, #5845, .T. ) ;
#6797=LINE ( 'NONE', #6643, #7863 ) ;
#6798=AXIS2_PLACEMENT_3D ( 'NONE', #687, #9083, #9293 ) ;
#6843=EDGE_CURVE ( 'NONE', #4689, #10017, #6389, .T. ) ;
#6956=CARTESIAN_POINT ( 'NONE',  ( 145.0000000000000284, -5.500000000000000000, 3.000000000000000000 ) ) ;
#6970=VERTEX_POINT ( 'NONE', #8567 ) ;
#6973=DIRECTION ( 'NONE',  ( 1.000000000000000000, 0.000000000000000000, 0.000000000000000000 ) ) ;
#6987=VECTOR ( 'NONE', #6164, 1000.000000000000000 ) ;
#7001=DIRECTION ( 'NONE',  ( 0.000000000000000000, -0.000000000000000000, -1.000000000000000000 ) ) ;
#7012=ORIENTED_EDGE ( 'NONE', *, *, #7089, .T. ) ;
#7044=ADVANCED_FACE ( 'NONE', ( #11 ), #5952, .F. ) ;
#7050=CARTESIAN_POINT ( 'NONE',  ( -149.9999999999999716, 8.000000000000000000, 0.000000000000000000 ) ) ;
#7089=EDGE_CURVE ( 'NONE', #427, #4976, #5565, .T. ) ;
#7116=FACE_OUTER_BOUND ( 'NONE', #814, .T. ) ;
#7129=DIRECTION ( 'NONE',  ( 1.000000000000000000, 0.000000000000000000, 0.000000000000000000 ) ) ;
#7136=EDGE_LOOP ( 'NONE', ( #1570, #3298 ) ) ;
#7147=VECTOR ( 'NONE', #7469, 1000.000000000000000 ) ;
#7156=VERTEX_POINT ( 'NONE', #6347 ) ;
#7163=CARTESIAN_POINT ( 'NONE',  ( -139.9999999999999716, -8.000000000000000000, 3.000000000000000000 ) ) ;
#7171=DIRECTION ( 'NONE',  ( 1.000000000000000000, 0.000000000000000000, 0.000000000000000000 ) ) ;
#7174=LINE ( 'NONE', #1110, #10613 ) ;
#7181=CARTESIAN_POINT ( 'NONE',  ( 150.0000000000000284, 2.500000000000000000, 2.000000000000000000 ) ) ;
#7191=ORIENTED_EDGE ( 'NONE', *, *, #4985, .F. ) ;
#7198=LINE ( 'NONE', #477, #1656 ) ;
#7202=ORIENTED_EDGE ( 'NONE', *, *, #7761, .T. ) ;
#7225=CARTESIAN_POINT ( 'NONE',  ( -149.9999999999999716, 8.000000000000000000, 3.000000000000000000 ) ) ;
#7253=CARTESIAN_POINT ( 'NONE',  ( -149.9999999999999716, -12.99999999999998757, 3.000000000000000000 ) ) ;
#7267=ORIENTED_EDGE ( 'NONE', *, *, #1779, .T. ) ;
#7274=EDGE_CURVE ( 'NONE', #2234, #767, #667, .T. ) ;
#7278=VECTOR ( 'NONE', #1341, 1000.000000000000000 ) ;
#7279=FACE_OUTER_BOUND ( 'NONE', #3266, .T. ) ;
#7283=VERTEX_POINT ( 'NONE', #7504 ) ;
#7287=VECTOR ( 'NONE', #8722, 1000.000000000000000 ) ;
#7328=PRODUCT ( 'stationary jaw', 'stationary jaw', '', ( #5143 ) ) ;
#7331=STYLED_ITEM('',(#11006),#1321);
#7373=DIRECTION ( 'NONE',  ( 0.000000000000000000, 0.000000000000000000, -1.000000000000000000 ) ) ;
#7389=ORIENTED_EDGE ( 'NONE', *, *, #3824, .T. ) ;
#7412=CARTESIAN_POINT ( 'NONE',  ( -105.0000000000000000, -2.500000000000000000, 3.000000000000000000 ) ) ;
#7420=EDGE_LOOP ( 'NONE', ( #8853, #6324, #9218, #10203 ) ) ;
#7429=ADVANCED_FACE ( 'NONE', ( #10257 ), #9323, .F. ) ;
#7441=VECTOR ( 'NONE', #6000, 1000.000000000000000 ) ;
#7455=CARTESIAN_POINT ( 'NONE',  ( 150.0000000000000284, -8.000000000000000000, 0.000000000000000000 ) ) ;
#7469=DIRECTION ( 'NONE',  ( -0.000000000000000000, -1.000000000000000000, -0.000000000000000000 ) ) ;
#7471=FACE_OUTER_BOUND ( 'NONE', #409, .T. ) ;
#7488=DIRECTION ( 'NONE',  ( 1.000000000000000000, 0.000000000000000000, 0.000000000000000000 ) ) ;
#7504=CARTESIAN_POINT ( 'NONE',  ( -144.9999999999999716, 33.00000000000000000, 3.000000000000000000 ) ) ;
#7540=LINE ( 'NONE', #3309, #4587 ) ;
#7614=VECTOR ( 'NONE', #4897, 1000.000000000000000 ) ;
#7627=DIRECTION ( 'NONE',  ( -1.000000000000000000, -0.000000000000000000, -0.000000000000000000 ) ) ;
#7643=CARTESIAN_POINT ( 'NONE',  ( 145.0000000000000284, 5.500000000000000000, 3.000000000000000000 ) ) ;
#7649=ORIENTED_EDGE ( 'NONE', *, *, #3757, .T. ) ;
#7653=PRESENTATION_STYLE_ASSIGNMENT (( #1876 ) ) ;
#7670=CARTESIAN_POINT ( 'NONE',  ( -144.9999999999999432, 8.000000000000000000, 3.000000000000000000 ) ) ;
#7699=EDGE_CURVE ( 'NONE', #767, #6540, #5487, .T. ) ;
#7705=DIRECTION ( 'NONE',  ( -0.000000000000000000, -0.000000000000000000, -1.000000000000000000 ) ) ;
#7712=SHAPE_REPRESENTATION_RELATIONSHIP ( 'NONE' , 'NONE' ,  #5016, #6551 ) ;
#7720=VERTEX_POINT ( 'NONE', #1940 ) ;
#7723=VERTEX_POINT ( 'NONE', #1998 ) ;
#7728=PLANE ( 'NONE',  #4205 ) ;
#7748=CARTESIAN_POINT ( 'NONE',  ( -105.0000000000000000, 2.500000000000000000, 2.000000000000000000 ) ) ;
#7761=EDGE_CURVE ( 'NONE', #6183, #2429, #6559, .T. ) ;
#7773=ORIENTED_EDGE ( 'NONE', *, *, #146, .F. ) ;
#7783=DIRECTION ( 'NONE',  ( -1.000000000000000000, 0.000000000000000000, 0.000000000000000000 ) ) ;
#7863=VECTOR ( 'NONE', #7627, 1000.000000000000000 ) ;
#7866=DIRECTION ( 'NONE',  ( -0.000000000000000000, -0.000000000000000000, 1.000000000000000000 ) ) ;
#7871=VERTEX_POINT ( 'NONE', #6454 ) ;
#7898=DIRECTION ( 'NONE',  ( -0.000000000000000000, -0.000000000000000000, 1.000000000000000000 ) ) ;
#7973=AXIS2_PLACEMENT_3D ( 'NONE', #5036, #2492, #5142 ) ;
#7979=VECTOR ( 'NONE', #5948, 1000.000000000000000 ) ;
#7985=EDGE_CURVE ( 'NONE', #9736, #9380, #9583, .T. ) ;
#8007=PLANE ( 'NONE',  #9442 ) ;
#8042=ORIENTED_EDGE ( 'NONE', *, *, #1779, .F. ) ;
#8054=CIRCLE ( 'NONE', #4301, 1.000000000000000888 ) ;
#8081=DIRECTION ( 'NONE',  ( 0.000000000000000000, -0.000000000000000000, 1.000000000000000000 ) ) ;
#8117=ORIENTED_EDGE ( 'NONE', *, *, #6408, .F. ) ;
#8148=( LENGTH_UNIT ( ) NAMED_UNIT ( * ) SI_UNIT ( .MILLI., .METRE. ) );
#8149=ORIENTED_EDGE ( 'NONE', *, *, #7089, .F. ) ;
#8161=VECTOR ( 'NONE', #10330, 1000.000000000000000 ) ;
#8218=AXIS2_PLACEMENT_3D ( 'NONE', #6465, #404, #4500 ) ;
#8275=ORIENTED_EDGE ( 'NONE', *, *, #1317, .F. ) ;
#8280=CARTESIAN_POINT ( 'NONE',  ( 150.0000000000000284, -8.000000000000000000, 3.000000000000000000 ) ) ;
#8298=FACE_OUTER_BOUND ( 'NONE', #5967, .T. ) ;
#8313=ORIENTED_EDGE ( 'NONE', *, *, #1429, .F. ) ;
#8331=ADVANCED_FACE ( 'NONE', ( #3047 ), #6494, .F. ) ;
#8386=( GEOMETRIC_REPRESENTATION_CONTEXT ( 3 ) GLOBAL_UNCERTAINTY_ASSIGNED_CONTEXT ( ( #1170 ) ) GLOBAL_UNIT_ASSIGNED_CONTEXT ( ( #8148, #1369, #2978 ) ) REPRESENTATION_CONTEXT ( 'NONE', 'WORKASPACE' ) );
#8407=ORIENTED_EDGE ( 'NONE', *, *, #4985, .T. ) ;
#8408=VECTOR ( 'NONE', #883, 1000.000000000000000 ) ;
#8438=ORIENTED_EDGE ( 'NONE', *, *, #9482, .F. ) ;
#8443=ADVANCED_FACE ( 'NONE', ( #1334 ), #8942, .T. ) ;
#8474=DIRECTION ( 'NONE',  ( -0.000000000000000000, -0.000000000000000000, -1.000000000000000000 ) ) ;
#8479=ORIENTED_EDGE ( 'NONE', *, *, #2918, .F. ) ;
#8526=FACE_OUTER_BOUND ( 'NONE', #10697, .T. ) ;
#8538=DIRECTION ( 'NONE',  ( 0.000000000000000000, 0.000000000000000000, -1.000000000000000000 ) ) ;
#8547=ORIENTED_EDGE ( 'NONE', *, *, #1671, .F. ) ;
#8567=CARTESIAN_POINT ( 'NONE',  ( -149.9999999999999716, 8.000000000000000000, 3.000000000000000000 ) ) ;
#8645=ORIENTED_EDGE ( 'NONE', *, *, #7274, .F. ) ;
#8656=ORIENTED_EDGE ( 'NONE', *, *, #2073, .F. ) ;
#8674=VECTOR ( 'NONE', #5531, 1000.000000000000000 ) ;
#8675=DIRECTION ( 'NONE',  ( -1.000000000000000000, 0.000000000000000000, -0.000000000000000000 ) ) ;
#8679=EDGE_CURVE ( 'NONE', #2164, #5869, #10789, .T. ) ;
#8693=DIRECTION ( 'NONE',  ( -0.000000000000000000, -0.000000000000000000, 1.000000000000000000 ) ) ;
#8695=CYLINDRICAL_SURFACE ( 'NONE', #599, 1.000000000000000888 ) ;
#8713=ADVANCED_FACE ( 'NONE', ( #10354 ), #5233, .F. ) ;
#8722=DIRECTION ( 'NONE',  ( -1.000000000000000000, -0.000000000000000000, -0.000000000000000000 ) ) ;
#8762=VECTOR ( 'NONE', #10350, 1000.000000000000000 ) ;
#8789=DIRECTION ( 'NONE',  ( 1.110223024625156540E-15, -1.000000000000000000, -0.000000000000000000 ) ) ;
#8802=ORIENTED_EDGE ( 'NONE', *, *, #6767, .F. ) ;
#8853=ORIENTED_EDGE ( 'NONE', *, *, #3539, .F. ) ;
#8876=AXIS2_PLACEMENT_3D ( 'NONE', #313, #2651, #4350 ) ;
#8893=CARTESIAN_POINT ( 'NONE',  ( -144.9999999999999432, 8.000000000000000000, 0.000000000000000000 ) ) ;
#8930=ORIENTED_EDGE ( 'NONE', *, *, #6269, .T. ) ;
#8936=AXIS2_PLACEMENT_3D ( 'NONE', #4806, #3983, #7373 ) ;
#8942=CYLINDRICAL_SURFACE ( 'NONE', #6349, 50.00000000000000000 ) ;
#8963=CARTESIAN_POINT ( 'NONE',  ( 150.0000000000000284, -8.000000000000000000, 2.000000000000000000 ) ) ;
#8979=ORIENTED_EDGE ( 'NONE', *, *, #7699, .F. ) ;
#9017=DIRECTION ( 'NONE',  ( -0.000000000000000000, -1.000000000000000000, -0.000000000000000000 ) ) ;
#9036=FACE_OUTER_BOUND ( 'NONE', #1774, .T. ) ;
#9038=VECTOR ( 'NONE', #3418, 1000.000000000000000 ) ;
#9045=VERTEX_POINT ( 'NONE', #731 ) ;
#9051=ORIENTED_EDGE ( 'NONE', *, *, #1587, .F. ) ;
#9083=DIRECTION ( 'NONE',  ( -1.000000000000000000, -1.734723475976807094E-15, 0.000000000000000000 ) ) ;
#9105=CARTESIAN_POINT ( 'NONE',  ( 150.0000000000000284, -8.000000000000000000, 3.000000000000000000 ) ) ;
#9134=DIRECTION ( 'NONE',  ( -0.000000000000000000, -0.000000000000000000, -1.000000000000000000 ) ) ;
#9143=PLANE ( 'NONE',  #8936 ) ;
#9155=PLANE ( 'NONE',  #1936 ) ;
#9178=LINE ( 'NONE', #2157, #8674 ) ;
#9186=CARTESIAN_POINT ( 'NONE',  ( 0.000000000000000000, 0.000000000000000000, 3.000000000000000000 ) ) ;
#9188=ADVANCED_FACE ( 'NONE', ( #9385 ), #7728, .T. ) ;
#9213=EDGE_CURVE ( 'NONE', #10197, #6498, #991, .T. ) ;
#9218=ORIENTED_EDGE ( 'NONE', *, *, #6350, .T. ) ;
#9228=ORIENTED_EDGE ( 'NONE', *, *, #1587, .T. ) ;
#9229=CARTESIAN_POINT ( 'NONE',  ( -134.9999999999999147, 8.000000000000000000, 0.000000000000000000 ) ) ;
#9238=CARTESIAN_POINT ( 'NONE',  ( 146.0000000000000284, 5.500000000000000000, 3.000000000000000000 ) ) ;
#9242=DIRECTION ( 'NONE',  ( -1.000000000000000000, 0.000000000000000000, -0.000000000000000000 ) ) ;
#9293=DIRECTION ( 'NONE',  ( 1.734723475976807094E-15, -1.000000000000000000, 0.000000000000000000 ) ) ;
#9319=EDGE_CURVE ( 'NONE', #9377, #6183, #3661, .T. ) ;
#9323=PLANE ( 'NONE',  #547 ) ;
#9339=DIRECTION ( 'NONE',  ( -0.000000000000000000, -0.000000000000000000, 1.000000000000000000 ) ) ;
#9350=CARTESIAN_POINT ( 'NONE',  ( 145.0000000000000284, -5.500000000000000000, 0.000000000000000000 ) ) ;
#9352=AXIS2_PLACEMENT_3D ( 'NONE', #9876, #3930, #2992 ) ;
#9356=CARTESIAN_POINT ( 'NONE',  ( 146.0000000000000284, -5.500000000000000000, 3.000000000000000000 ) ) ;
#9359=EDGE_CURVE ( 'NONE', #2994, #3747, #328, .T. ) ;
#9363=CARTESIAN_POINT ( 'NONE',  ( 0.000000000000000000, 0.000000000000000000, 0.000000000000000000 ) ) ;
#9377=VERTEX_POINT ( 'NONE', #2955 ) ;
#9380=VERTEX_POINT ( 'NONE', #2062 ) ;
#9383=LINE ( 'NONE', #53, #8408 ) ;
#9385=FACE_OUTER_BOUND ( 'NONE', #3735, .T. ) ;
#9388=CARTESIAN_POINT ( 'NONE',  ( 150.0000000000000284, -2.500000000000000444, 3.000000000000000000 ) ) ;
#9392=VERTEX_POINT ( 'NONE', #9671 ) ;
#9393=CARTESIAN_POINT ( 'NONE',  ( -149.9999999999999716, -8.000000000000000000, 3.000000000000000000 ) ) ;
#9424=SURFACE_STYLE_FILL_AREA ( #4419 ) ;
#9426=VECTOR ( 'NONE', #2563, 1000.000000000000000 ) ;
#9442=AXIS2_PLACEMENT_3D ( 'NONE', #7225, #2115, #7001 ) ;
#9445=CARTESIAN_POINT ( 'NONE',  ( -139.9999999999999716, -43.00000000000000000, 0.000000000000000000 ) ) ;
#9465=DIRECTION ( 'NONE',  ( -0.000000000000000000, -0.000000000000000000, 1.000000000000000000 ) ) ;
#9482=EDGE_CURVE ( 'NONE', #10003, #6970, #2176, .T. ) ;
#9505=CARTESIAN_POINT ( 'NONE',  ( 150.0000000000000000, 2.500000000000000444, 3.000000000000000000 ) ) ;
#9531=VERTEX_POINT ( 'NONE', #3114 ) ;
#9536=( NAMED_UNIT ( * ) SI_UNIT ( $, .STERADIAN. ) SOLID_ANGLE_UNIT ( ) );
#9571=ORIENTED_EDGE ( 'NONE', *, *, #9639, .F. ) ;
#9583=CIRCLE ( 'NONE', #2482, 50.00000000000000000 ) ;
#9606=ORIENTED_EDGE ( 'NONE', *, *, #9213, .F. ) ;
#9624=ORIENTED_EDGE ( 'NONE', *, *, #4304, .F. ) ;
#9639=EDGE_CURVE ( 'NONE', #5859, #7720, #10619, .T. ) ;
#9648=AXIS2_PLACEMENT_3D ( 'NONE', #9350, #8693, #10286 ) ;
#9662=ORIENTED_EDGE ( 'NONE', *, *, #6711, .T. ) ;
#9671=CARTESIAN_POINT ( 'NONE',  ( 146.0000000000000284, -5.500000000000000000, 0.000000000000000000 ) ) ;
#9674=LINE ( 'NONE', #10443, #150 ) ;
#9696=EDGE_CURVE ( 'NONE', #192, #1190, #2544, .T. ) ;
#9707=EDGE_LOOP ( 'NONE', ( #1751, #1162, #6722, #7267 ) ) ;
#9732=ADVANCED_FACE ( 'NONE', ( #10312 ), #2714, .F. ) ;
#9733=UNCERTAINTY_MEASURE_WITH_UNIT (LENGTH_MEASURE( 1.000000000000000082E-05 ), #5978, 'distance_accuracy_value', 'NONE');
#9736=VERTEX_POINT ( 'NONE', #4536 ) ;
#9769=VECTOR ( 'NONE', #406, 1000.000000000000000 ) ;
#9778=LINE ( 'NONE', #8893, #4826 ) ;
#9806=DIRECTION ( 'NONE',  ( 1.000000000000000000, -0.000000000000000000, 0.000000000000000000 ) ) ;
#9808=ORIENTED_EDGE ( 'NONE', *, *, #2266, .T. ) ;
#9826=CARTESIAN_POINT ( 'NONE',  ( -99.99999999999995737, -12.99999999999998757, 3.000000000000000000 ) ) ;
#9830=VECTOR ( 'NONE', #4822, 1000.000000000000000 ) ;
#9837=EDGE_CURVE ( 'NONE', #9380, #9377, #5249, .T. ) ;
#9841=CARTESIAN_POINT ( 'NONE',  ( -139.9999999999999716, -8.000000000000000000, 3.000000000000000000 ) ) ;
#9870=ORIENTED_EDGE ( 'NONE', *, *, #10917, .F. ) ;
#9876=CARTESIAN_POINT ( 'NONE',  ( -139.9999999999999716, -8.000000000000000000, 3.000000000000000000 ) ) ;
#9882=CARTESIAN_POINT ( 'NONE',  ( -144.9999999999999432, 8.000000000000000000, 3.000000000000000000 ) ) ;
#9935=STYLED_ITEM ( 'NONE', ( #7653 ), #6551 ) ;
#9945=DIRECTION ( 'NONE',  ( 1.000000000000000000, 0.000000000000000000, 0.000000000000000000 ) ) ;
#9969=LINE ( 'NONE', #2252, #7614 ) ;
#9980=ADVANCED_FACE ( 'NONE', ( #1438 ), #4814, .F. ) ;
#9991=ORIENTED_EDGE ( 'NONE', *, *, #5725, .T. ) ;
#10003=VERTEX_POINT ( 'NONE', #9882 ) ;
#10007=CARTESIAN_POINT ( 'NONE',  ( 144.0000000000000284, -5.500000000000000000, 3.000000000000000000 ) ) ;
#10016=FACE_OUTER_BOUND ( 'NONE', #6271, .T. ) ;
#10017=VERTEX_POINT ( 'NONE', #2321 ) ;
#10048=EDGE_LOOP ( 'NONE', ( #6524, #9051, #2225, #10151 ) ) ;
#10063=ORIENTED_EDGE ( 'NONE', *, *, #1671, .T. ) ;
#10075=VECTOR ( 'NONE', #9017, 1000.000000000000000 ) ;
#10120=ORIENTED_EDGE ( 'NONE', *, *, #9319, .F. ) ;
#10151=ORIENTED_EDGE ( 'NONE', *, *, #7699, .T. ) ;
#10152=CARTESIAN_POINT ( 'NONE',  ( -144.9999999999999432, 8.000000000000000000, 3.000000000000000000 ) ) ;
#10159=CARTESIAN_POINT ( 'NONE',  ( 0.000000000000000000, 2.500000000000000000, 3.000000000000000000 ) ) ;
#10183=DIRECTION ( 'NONE',  ( -0.000000000000000000, -0.000000000000000000, 1.000000000000000000 ) ) ;
#10197=VERTEX_POINT ( 'NONE', #4188 ) ;
#10203=ORIENTED_EDGE ( 'NONE', *, *, #6711, .F. ) ;
#10228=EDGE_LOOP ( 'NONE', ( #8042, #10934 ) ) ;
#10235=LINE ( 'NONE', #4979, #10709 ) ;
#10237=CARTESIAN_POINT ( 'NONE',  ( 150.0000000000000284, -8.000000000000000000, 3.000000000000000000 ) ) ;
#10257=FACE_OUTER_BOUND ( 'NONE', #5479, .T. ) ;
#10258=AXIS2_PLACEMENT_3D ( 'NONE', #1952, #4549, #3727 ) ;
#10286=DIRECTION ( 'NONE',  ( 1.000000000000000000, 0.000000000000000000, 0.000000000000000000 ) ) ;
#10290=EDGE_CURVE ( 'NONE', #6091, #767, #7540, .T. ) ;
#10292=CARTESIAN_POINT ( 'NONE',  ( 145.0000000000000284, 5.500000000000000000, 3.000000000000000000 ) ) ;
#10302=PRODUCT_DEFINITION ( 'UNKNOWN', '', #5499, #5604 ) ;
#10308=SURFACE_SIDE_STYLE ('',( #9424 ) ) ;
#10309=ORIENTED_EDGE ( 'NONE', *, *, #1317, .T. ) ;
#10312=FACE_OUTER_BOUND ( 'NONE', #2748, .T. ) ;
#10330=DIRECTION ( 'NONE',  ( 0.000000000000000000, 0.000000000000000000, -1.000000000000000000 ) ) ;
#10335=DIRECTION ( 'NONE',  ( 1.000000000000000000, 0.000000000000000000, 0.000000000000000000 ) ) ;
#10337=DIRECTION ( 'NONE',  ( 1.000000000000000000, 0.000000000000000000, 0.000000000000000000 ) ) ;
#10339=VECTOR ( 'NONE', #5519, 1000.000000000000000 ) ;
#10350=DIRECTION ( 'NONE',  ( -1.000000000000000000, -0.000000000000000000, -0.000000000000000000 ) ) ;
#10354=FACE_OUTER_BOUND ( 'NONE', #9707, .T. ) ;
#10369=ORIENTED_EDGE ( 'NONE', *, *, #5877, .F. ) ;
#10390=EDGE_LOOP ( 'NONE', ( #8438, #2114, #8930, #8802 ) ) ;
#10434=CARTESIAN_POINT ( 'NONE',  ( -149.9999999999999716, -8.000000000000000000, 3.000000000000000000 ) ) ;
#10443=CARTESIAN_POINT ( 'NONE',  ( -144.9999999999999432, 8.000000000000000000, 3.000000000000000000 ) ) ;
#10451=VECTOR ( 'NONE', #762, 1000.000000000000000 ) ;
#10464=ORIENTED_EDGE ( 'NONE', *, *, #2830, .T. ) ;
#10471=ORIENTED_EDGE ( 'NONE', *, *, #4038, .T. ) ;
#10485=DIRECTION ( 'NONE',  ( 0.000000000000000000, -0.000000000000000000, 1.000000000000000000 ) ) ;
#10495=FACE_OUTER_BOUND ( 'NONE', #10390, .T. ) ;
#10525=VECTOR ( 'NONE', #7866, 1000.000000000000000 ) ;
#10548=EDGE_CURVE ( 'NONE', #7156, #6540, #9178, .T. ) ;
#10556=DIRECTION ( 'NONE',  ( -0.000000000000000000, -0.000000000000000000, -1.000000000000000000 ) ) ;
#10570=EDGE_CURVE ( 'NONE', #5859, #9531, #4698, .T. ) ;
#10594=DIRECTION ( 'NONE',  ( 1.000000000000000000, 0.000000000000000000, 0.000000000000000000 ) ) ;
#10613=VECTOR ( 'NONE', #4663, 1000.000000000000000 ) ;
#10619=CIRCLE ( 'NONE', #7973, 50.00000000000000000 ) ;
#10662=CYLINDRICAL_SURFACE ( 'NONE', #2825, 1.000000000000000888 ) ;
#10665=EDGE_CURVE ( 'NONE', #2429, #4976, #3385, .T. ) ;
#10692=EDGE_CURVE ( 'NONE', #6498, #7723, #4267, .T. ) ;
#10695=ORIENTED_EDGE ( 'NONE', *, *, #1280, .T. ) ;
#10697=EDGE_LOOP ( 'NONE', ( #6533, #6428, #9662, #1033 ) ) ;
#10699=VECTOR ( 'NONE', #6675, 1000.000000000000000 ) ;
#10709=VECTOR ( 'NONE', #4465, 1000.000000000000000 ) ;
#10724=ORIENTED_EDGE ( 'NONE', *, *, #10570, .T. ) ;
#10748=FACE_BOUND ( 'NONE', #10228, .T. ) ;
#10763=CARTESIAN_POINT ( 'NONE',  ( -149.9999999999999716, 8.000000000000000000, 3.000000000000000000 ) ) ;
#10789=CIRCLE ( 'NONE', #678, 1.000000000000000888 ) ;
#10867=CIRCLE ( 'NONE', #1482, 30.00000000000000000 ) ;
#10872=APPLICATION_CONTEXT ( 'automotive_design' ) ;
#10873=EDGE_LOOP ( 'NONE', ( #4403, #10369, #4704, #3529 ) ) ;
#10917=EDGE_CURVE ( 'NONE', #7283, #10003, #9674, .T. ) ;
#10923=ORIENTED_EDGE ( 'NONE', *, *, #10692, .T. ) ;
#10934=ORIENTED_EDGE ( 'NONE', *, *, #8679, .F. ) ;
#10948=CARTESIAN_POINT ( 'NONE',  ( 145.0000000000000284, 5.500000000000000000, 0.000000000000000000 ) ) ;
#11000=COLOUR_RGB('Light Blue',0.38,0.62,0.78);
#11001=FILL_AREA_STYLE_COLOUR('',#11000);
#11002=FILL_AREA_STYLE('',(#11001));
#11003=SURFACE_STYLE_FILL_AREA(#11002);
#11004=SURFACE_SIDE_STYLE('',(#11003));
#11005=SURFACE_STYLE_USAGE(.BOTH.,#11004);
#11006=PRESENTATION_STYLE_ASSIGNMENT((#11005));
ENDSEC;
END-ISO-10303-21;
